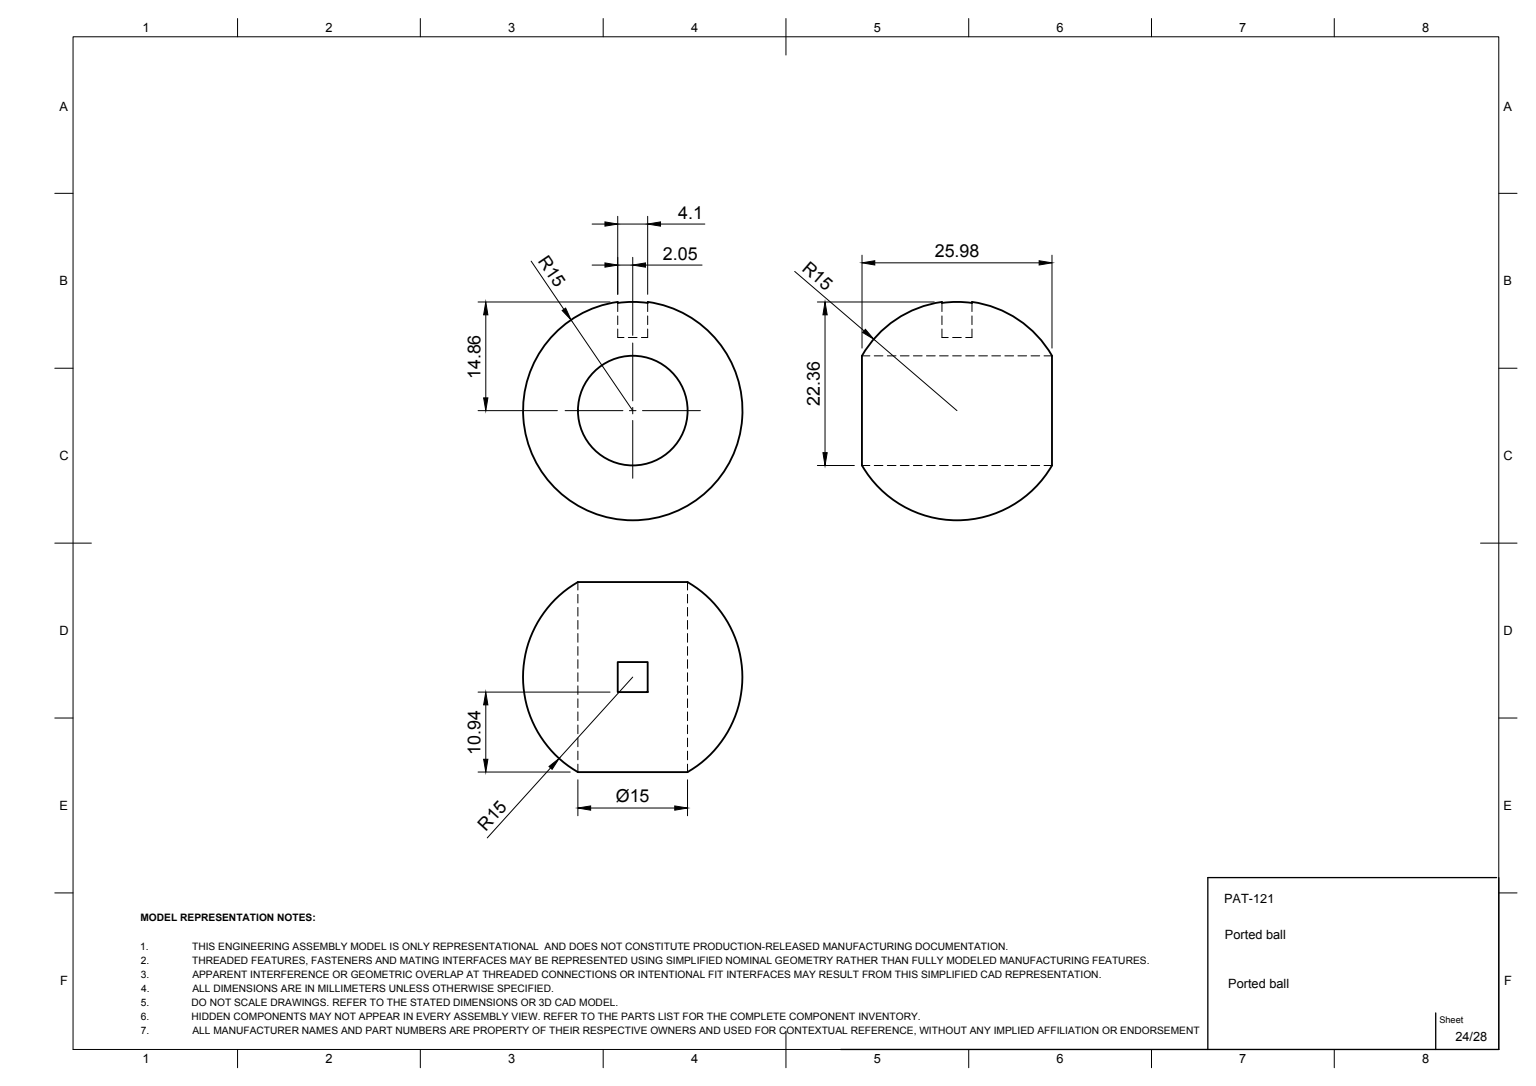
ISO-10303-21;
HEADER;
/* Generated by software containing ST-Developer
 * from STEP Tools, Inc. (www.steptools.com) 
 */

FILE_DESCRIPTION(
/* description */ ('Wall-mounted air drop station'),
/* implementation_level */ '2;1');

FILE_NAME(
/* name */ 'Ported ball.step',
/* time_stamp */ '2026-10-28T22:16:19-07:00',
/* author */ (''),
/* organization */ (''),
/* preprocessor_version */ 'ST-DEVELOPER v20.2',
/* originating_system */ 'Autodesk Translation Framework v15.17.0.0',
/* authorisation */ '');

FILE_SCHEMA (('AUTOMOTIVE_DESIGN { 1 0 10303 214 3 1 1 }'));
ENDSEC;

DATA;
#10=MECHANICAL_DESIGN_GEOMETRIC_PRESENTATION_REPRESENTATION('',(#367),#10517);
#263=SPHERICAL_SURFACE('',#6828,1.5);
#309=SHAPE_REPRESENTATION_RELATIONSHIP('SRR','None',#10667,#338);
#338=ADVANCED_BREP_SHAPE_REPRESENTATION('',(#394),#10511);
#367=STYLED_ITEM('',(#10860),#394);
#394=MANIFOLD_SOLID_BREP('Body1',#5908);
#517=FACE_BOUND('',#1525,.T.);
#518=FACE_BOUND('',#1526,.T.);
#701=PLANE('',#6815);
#702=PLANE('',#6817);
#703=PLANE('',#6820);
#704=PLANE('',#6822);
#705=PLANE('',#6824);
#1045=FACE_OUTER_BOUND('',#1518,.T.);
#1046=FACE_OUTER_BOUND('',#1519,.T.);
#1047=FACE_OUTER_BOUND('',#1520,.T.);
#1048=FACE_OUTER_BOUND('',#1521,.T.);
#1049=FACE_OUTER_BOUND('',#1522,.T.);
#1050=FACE_OUTER_BOUND('',#1523,.T.);
#1051=FACE_OUTER_BOUND('',#1524,.T.);
#1518=EDGE_LOOP('',(#5161,#5162,#5163,#5164));
#1519=EDGE_LOOP('',(#5165,#5166,#5167,#5168,#5169));
#1520=EDGE_LOOP('',(#5170,#5171,#5172,#5173));
#1521=EDGE_LOOP('',(#5174,#5175,#5176,#5177));
#1522=EDGE_LOOP('',(#5178,#5179,#5180,#5181));
#1523=EDGE_LOOP('',(#5182,#5183,#5184,#5185));
#1524=EDGE_LOOP('',(#5186,#5187,#5188,#5189,#5190,#5191,#5192));
#1525=EDGE_LOOP('',(#5193));
#1526=EDGE_LOOP('',(#5194));
#1952=LINE('',#10157,#2416);
#1953=LINE('',#10159,#2417);
#1954=LINE('',#10160,#2418);
#1955=LINE('',#10165,#2419);
#1956=LINE('',#10167,#2420);
#1957=LINE('',#10173,#2421);
#1958=LINE('',#10174,#2422);
#1959=LINE('',#10177,#2423);
#1960=LINE('',#10183,#2424);
#2416=VECTOR('',#8448,1.);
#2417=VECTOR('',#8449,1.);
#2418=VECTOR('',#8450,1.);
#2419=VECTOR('',#8455,1.);
#2420=VECTOR('',#8456,1.);
#2421=VECTOR('',#8463,1.);
#2422=VECTOR('',#8464,1.);
#2423=VECTOR('',#8469,1.);
#2424=VECTOR('',#8476,0.75);
#2734=CIRCLE('',#6816,1.48592563743951);
#2735=CIRCLE('',#6818,1.48592563743951);
#2736=CIRCLE('',#6819,1.48592563743951);
#2737=CIRCLE('',#6821,1.48592563743951);
#2738=CIRCLE('',#6823,1.48592563743951);
#2739=CIRCLE('',#6826,0.75);
#2740=CIRCLE('',#6827,0.75);
#2741=CIRCLE('',#6829,1.5);
#3157=VERTEX_POINT('',#10153);
#3158=VERTEX_POINT('',#10154);
#3159=VERTEX_POINT('',#10156);
#3160=VERTEX_POINT('',#10158);
#3161=VERTEX_POINT('',#10162);
#3162=VERTEX_POINT('',#10164);
#3163=VERTEX_POINT('',#10166);
#3164=VERTEX_POINT('',#10170);
#3165=VERTEX_POINT('',#10172);
#3166=VERTEX_POINT('',#10180);
#3167=VERTEX_POINT('',#10182);
#3168=VERTEX_POINT('',#10186);
#3838=EDGE_CURVE('',#3157,#3158,#2734,.T.);
#3839=EDGE_CURVE('',#3159,#3157,#1952,.T.);
#3840=EDGE_CURVE('',#3160,#3159,#1953,.T.);
#3841=EDGE_CURVE('',#3160,#3158,#1954,.T.);
#3842=EDGE_CURVE('',#3158,#3161,#2735,.T.);
#3843=EDGE_CURVE('',#3162,#3160,#1955,.T.);
#3844=EDGE_CURVE('',#3162,#3163,#1956,.T.);
#3845=EDGE_CURVE('',#3161,#3163,#2736,.T.);
#3846=EDGE_CURVE('',#3163,#3164,#2737,.T.);
#3847=EDGE_CURVE('',#3165,#3162,#1957,.T.);
#3848=EDGE_CURVE('',#3165,#3164,#1958,.T.);
#3849=EDGE_CURVE('',#3164,#3157,#2738,.T.);
#3850=EDGE_CURVE('',#3159,#3165,#1959,.T.);
#3851=EDGE_CURVE('',#3166,#3166,#2739,.T.);
#3852=EDGE_CURVE('',#3166,#3167,#1960,.T.);
#3853=EDGE_CURVE('',#3167,#3167,#2740,.T.);
#3854=EDGE_CURVE('',#3161,#3168,#2741,.T.);
#5161=ORIENTED_EDGE('',*,*,#3838,.F.);
#5162=ORIENTED_EDGE('',*,*,#3839,.F.);
#5163=ORIENTED_EDGE('',*,*,#3840,.F.);
#5164=ORIENTED_EDGE('',*,*,#3841,.T.);
#5165=ORIENTED_EDGE('',*,*,#3842,.F.);
#5166=ORIENTED_EDGE('',*,*,#3841,.F.);
#5167=ORIENTED_EDGE('',*,*,#3843,.F.);
#5168=ORIENTED_EDGE('',*,*,#3844,.T.);
#5169=ORIENTED_EDGE('',*,*,#3845,.F.);
#5170=ORIENTED_EDGE('',*,*,#3846,.F.);
#5171=ORIENTED_EDGE('',*,*,#3844,.F.);
#5172=ORIENTED_EDGE('',*,*,#3847,.F.);
#5173=ORIENTED_EDGE('',*,*,#3848,.T.);
#5174=ORIENTED_EDGE('',*,*,#3849,.F.);
#5175=ORIENTED_EDGE('',*,*,#3848,.F.);
#5176=ORIENTED_EDGE('',*,*,#3850,.F.);
#5177=ORIENTED_EDGE('',*,*,#3839,.T.);
#5178=ORIENTED_EDGE('',*,*,#3843,.T.);
#5179=ORIENTED_EDGE('',*,*,#3840,.T.);
#5180=ORIENTED_EDGE('',*,*,#3850,.T.);
#5181=ORIENTED_EDGE('',*,*,#3847,.T.);
#5182=ORIENTED_EDGE('',*,*,#3851,.F.);
#5183=ORIENTED_EDGE('',*,*,#3852,.T.);
#5184=ORIENTED_EDGE('',*,*,#3853,.F.);
#5185=ORIENTED_EDGE('',*,*,#3852,.F.);
#5186=ORIENTED_EDGE('',*,*,#3846,.T.);
#5187=ORIENTED_EDGE('',*,*,#3849,.T.);
#5188=ORIENTED_EDGE('',*,*,#3838,.T.);
#5189=ORIENTED_EDGE('',*,*,#3842,.T.);
#5190=ORIENTED_EDGE('',*,*,#3854,.T.);
#5191=ORIENTED_EDGE('',*,*,#3854,.F.);
#5192=ORIENTED_EDGE('',*,*,#3845,.T.);
#5193=ORIENTED_EDGE('',*,*,#3853,.T.);
#5194=ORIENTED_EDGE('',*,*,#3851,.T.);
#5521=CYLINDRICAL_SURFACE('',#6825,0.75);
#5818=ADVANCED_FACE('',(#1045),#701,.F.);
#5819=ADVANCED_FACE('',(#1046),#702,.F.);
#5820=ADVANCED_FACE('',(#1047),#703,.F.);
#5821=ADVANCED_FACE('',(#1048),#704,.F.);
#5822=ADVANCED_FACE('',(#1049),#705,.T.);
#5823=ADVANCED_FACE('',(#1050),#5521,.F.);
#5824=ADVANCED_FACE('',(#1051,#517,#518),#263,.T.);
#5908=CLOSED_SHELL('',(#5818,#5819,#5820,#5821,#5822,#5823,#5824));
#6814=AXIS2_PLACEMENT_3D('',#10151,#8442,#8443);
#6815=AXIS2_PLACEMENT_3D('',#10152,#8444,#8445);
#6816=AXIS2_PLACEMENT_3D('',#10155,#8446,#8447);
#6817=AXIS2_PLACEMENT_3D('',#10161,#8451,#8452);
#6818=AXIS2_PLACEMENT_3D('',#10163,#8453,#8454);
#6819=AXIS2_PLACEMENT_3D('',#10168,#8457,#8458);
#6820=AXIS2_PLACEMENT_3D('',#10169,#8459,#8460);
#6821=AXIS2_PLACEMENT_3D('',#10171,#8461,#8462);
#6822=AXIS2_PLACEMENT_3D('',#10175,#8465,#8466);
#6823=AXIS2_PLACEMENT_3D('',#10176,#8467,#8468);
#6824=AXIS2_PLACEMENT_3D('',#10178,#8470,#8471);
#6825=AXIS2_PLACEMENT_3D('',#10179,#8472,#8473);
#6826=AXIS2_PLACEMENT_3D('',#10181,#8474,#8475);
#6827=AXIS2_PLACEMENT_3D('',#10184,#8477,#8478);
#6828=AXIS2_PLACEMENT_3D('',#10185,#8479,#8480);
#6829=AXIS2_PLACEMENT_3D('',#10187,#8481,#8482);
#8442=DIRECTION('axis',(0.,0.,1.));
#8443=DIRECTION('refdir',(1.,0.,0.));
#8444=DIRECTION('center_axis',(0.,-1.,0.));
#8445=DIRECTION('ref_axis',(1.,0.,0.));
#8446=DIRECTION('center_axis',(0.,-1.,0.));
#8447=DIRECTION('ref_axis',(0.,0.,1.));
#8448=DIRECTION('',(0.,0.,1.));
#8449=DIRECTION('',(1.,0.,0.));
#8450=DIRECTION('',(0.,0.,1.));
#8451=DIRECTION('center_axis',(-1.,0.,0.));
#8452=DIRECTION('ref_axis',(0.,-1.,0.));
#8453=DIRECTION('center_axis',(-1.,0.,0.));
#8454=DIRECTION('ref_axis',(0.,0.,-1.));
#8455=DIRECTION('',(0.,-1.,0.));
#8456=DIRECTION('',(0.,0.,1.));
#8457=DIRECTION('center_axis',(-1.,0.,0.));
#8458=DIRECTION('ref_axis',(0.,0.,-1.));
#8459=DIRECTION('center_axis',(0.,1.,0.));
#8460=DIRECTION('ref_axis',(-1.,0.,0.));
#8461=DIRECTION('center_axis',(0.,1.,0.));
#8462=DIRECTION('ref_axis',(0.,0.,-1.));
#8463=DIRECTION('',(-1.,0.,0.));
#8464=DIRECTION('',(0.,0.,1.));
#8465=DIRECTION('center_axis',(1.,0.,0.));
#8466=DIRECTION('ref_axis',(0.,1.,0.));
#8467=DIRECTION('center_axis',(1.,0.,0.));
#8468=DIRECTION('ref_axis',(0.,0.,1.));
#8469=DIRECTION('',(0.,1.,0.));
#8470=DIRECTION('center_axis',(0.,0.,1.));
#8471=DIRECTION('ref_axis',(1.,0.,0.));
#8472=DIRECTION('center_axis',(0.,1.,0.));
#8473=DIRECTION('ref_axis',(1.,0.,0.));
#8474=DIRECTION('center_axis',(0.,1.,0.));
#8475=DIRECTION('ref_axis',(1.,0.,0.));
#8476=DIRECTION('',(0.,1.,0.));
#8477=DIRECTION('center_axis',(0.,-1.,0.));
#8478=DIRECTION('ref_axis',(1.,0.,0.));
#8479=DIRECTION('center_axis',(6.12323399573677E-17,0.,1.));
#8480=DIRECTION('ref_axis',(1.,0.,0.));
#8481=DIRECTION('center_axis',(1.22464679914735E-16,-1.,0.));
#8482=DIRECTION('ref_axis',(-1.,-1.22464679914735E-16,0.));
#10151=CARTESIAN_POINT('',(0.,0.,0.));
#10152=CARTESIAN_POINT('Origin',(-0.205,-0.205,6.));
#10153=CARTESIAN_POINT('',(0.205,-0.205,6.47171668469172));
#10154=CARTESIAN_POINT('',(-0.205,-0.205,6.47171668469172));
#10155=CARTESIAN_POINT('Origin',(0.,-0.205,5.));
#10156=CARTESIAN_POINT('',(0.205,-0.205,6.));
#10157=CARTESIAN_POINT('',(0.205,-0.205,6.));
#10158=CARTESIAN_POINT('',(-0.205,-0.205,6.));
#10159=CARTESIAN_POINT('',(-0.205,-0.205,6.));
#10160=CARTESIAN_POINT('',(-0.205,-0.205,6.));
#10161=CARTESIAN_POINT('Origin',(-0.205,0.205,6.));
#10162=CARTESIAN_POINT('',(-0.205,-2.51052593825207E-17,6.48592563743951));
#10163=CARTESIAN_POINT('Origin',(-0.205,0.,5.));
#10164=CARTESIAN_POINT('',(-0.205,0.205,6.));
#10165=CARTESIAN_POINT('',(-0.205,0.205,6.));
#10166=CARTESIAN_POINT('',(-0.205,0.205,6.47171668469172));
#10167=CARTESIAN_POINT('',(-0.205,0.205,6.));
#10168=CARTESIAN_POINT('Origin',(-0.205,0.,5.));
#10169=CARTESIAN_POINT('Origin',(0.205,0.205,6.));
#10170=CARTESIAN_POINT('',(0.205,0.205,6.47171668469172));
#10171=CARTESIAN_POINT('Origin',(0.,0.205,5.));
#10172=CARTESIAN_POINT('',(0.205,0.205,6.));
#10173=CARTESIAN_POINT('',(0.205,0.205,6.));
#10174=CARTESIAN_POINT('',(0.205,0.205,6.));
#10175=CARTESIAN_POINT('Origin',(0.205,-0.205,6.));
#10176=CARTESIAN_POINT('Origin',(0.205,0.,5.));
#10177=CARTESIAN_POINT('',(0.205,-0.205,6.));
#10178=CARTESIAN_POINT('Origin',(0.,0.,6.));
#10179=CARTESIAN_POINT('Origin',(0.,-1.6,5.));
#10180=CARTESIAN_POINT('',(-0.75,-1.29903810567666,5.));
#10181=CARTESIAN_POINT('Origin',(0.,-1.29903810567666,5.));
#10182=CARTESIAN_POINT('',(-0.75,1.29903810567666,5.));
#10183=CARTESIAN_POINT('',(-0.75,-1.6,5.));
#10184=CARTESIAN_POINT('Origin',(0.,1.29903810567666,5.));
#10185=CARTESIAN_POINT('Origin',(0.,0.,5.));
#10186=CARTESIAN_POINT('',(-9.18485099360515E-17,-1.12481983699639E-32,
3.5));
#10187=CARTESIAN_POINT('Origin',(0.,0.,5.));
#10478=UNCERTAINTY_MEASURE_WITH_UNIT(LENGTH_MEASURE(0.001),#10518,
'DISTANCE_ACCURACY_VALUE',
'Maximum model space distance between geometric entities at asserted c
onnectivities');
#10484=UNCERTAINTY_MEASURE_WITH_UNIT(LENGTH_MEASURE(0.001),#10518,
'DISTANCE_ACCURACY_VALUE',
'Maximum model space distance between geometric entities at asserted c
onnectivities');
#10511=(
GEOMETRIC_REPRESENTATION_CONTEXT(3)
GLOBAL_UNCERTAINTY_ASSIGNED_CONTEXT((#10478))
GLOBAL_UNIT_ASSIGNED_CONTEXT((#10518,#10520,#10521))
REPRESENTATION_CONTEXT('','3D')
);
#10517=(
GEOMETRIC_REPRESENTATION_CONTEXT(3)
GLOBAL_UNCERTAINTY_ASSIGNED_CONTEXT((#10484))
GLOBAL_UNIT_ASSIGNED_CONTEXT((#10518,#10520,#10521))
REPRESENTATION_CONTEXT('','3D')
);
#10518=(
LENGTH_UNIT()
NAMED_UNIT(*)
SI_UNIT(.CENTI.,.METRE.)
);
#10520=(
NAMED_UNIT(*)
PLANE_ANGLE_UNIT()
SI_UNIT($,.RADIAN.)
);
#10521=(
NAMED_UNIT(*)
SI_UNIT($,.STERADIAN.)
SOLID_ANGLE_UNIT()
);
#10548=SHAPE_DEFINITION_REPRESENTATION(#10627,#10667);
#10627=PRODUCT_DEFINITION_SHAPE('',$,#10700);
#10667=SHAPE_REPRESENTATION('',(#6814),#10511);
#10673=PRODUCT_DEFINITION_CONTEXT('part definition',#10771,'design');
#10700=PRODUCT_DEFINITION('Ported ball','Ported ball',#10732,#10673);
#10732=PRODUCT_DEFINITION_FORMATION('',$,#10799);
#10771=APPLICATION_CONTEXT(
'Core Data for Automotive Mechanical Design Process');
#10772=PRODUCT_CONTEXT('part definition',#10771,'mechanical');
#10799=PRODUCT('Ported ball','Ported ball','Ported ball',(#10772));
#10854=COLOUR_RGB('Light Blue',0.38,0.62,0.78);
#10855=FILL_AREA_STYLE_COLOUR('',#10854);
#10856=FILL_AREA_STYLE('',(#10855));
#10857=SURFACE_STYLE_FILL_AREA(#10856);
#10858=SURFACE_SIDE_STYLE('',(#10857));
#10859=SURFACE_STYLE_USAGE(.BOTH.,#10858);
#10860=PRESENTATION_STYLE_ASSIGNMENT((#10859));
ENDSEC;
END-ISO-10303-21;
